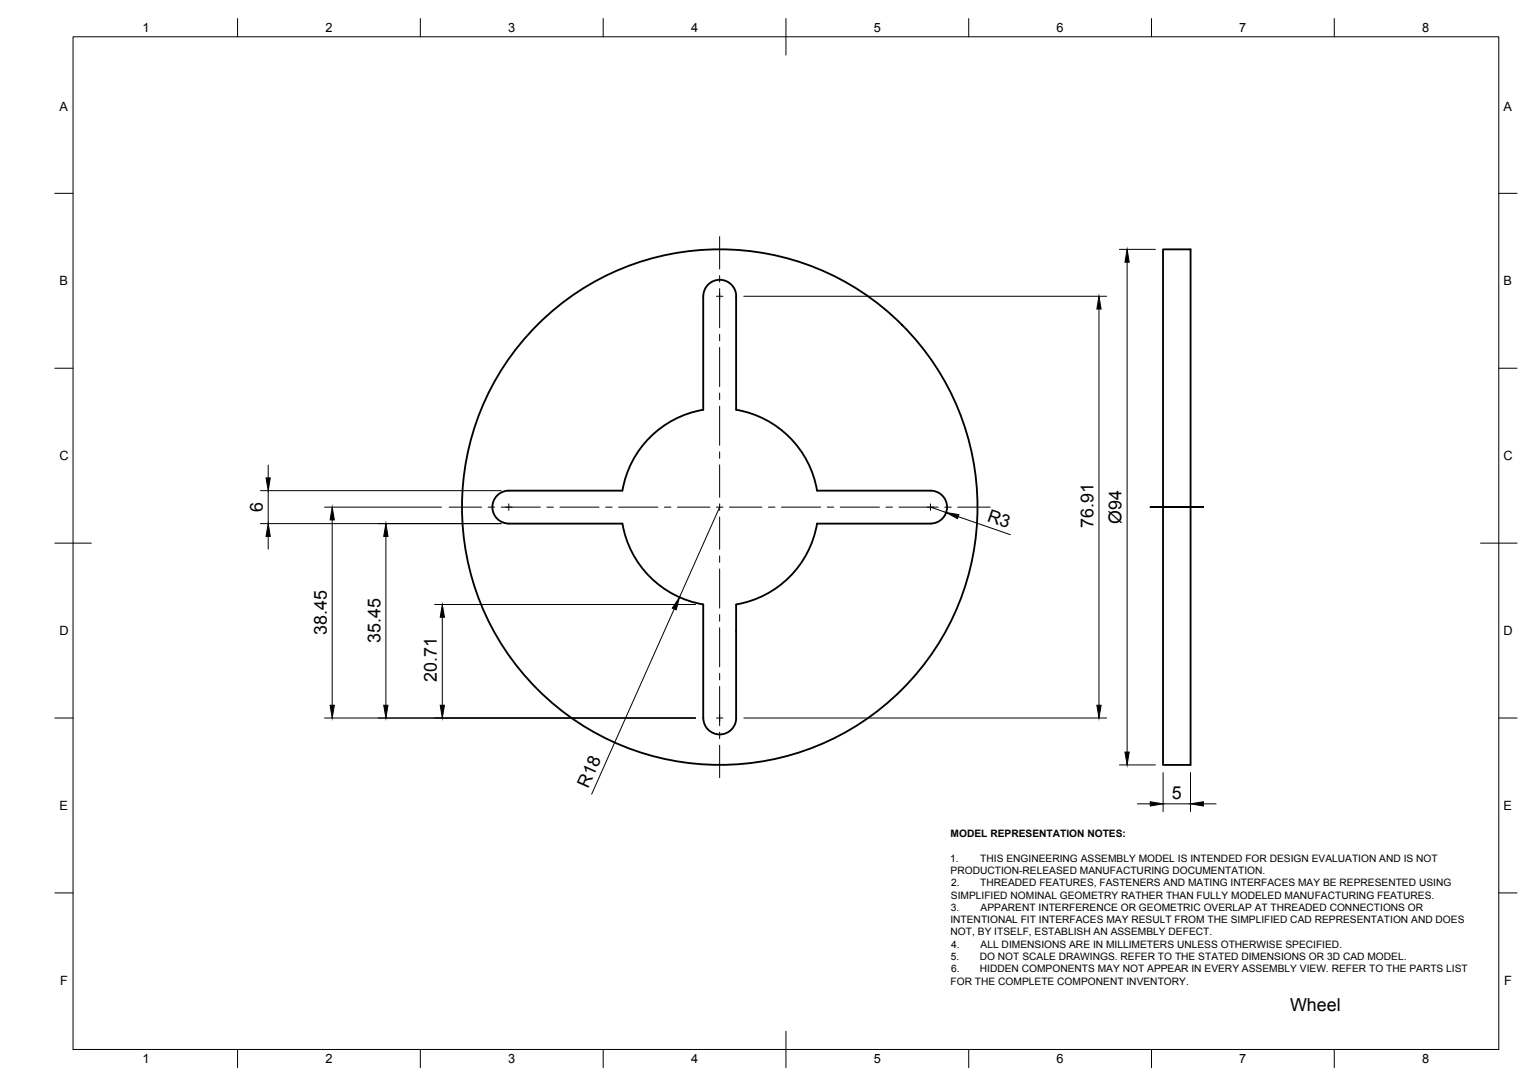
ISO-10303-21;
HEADER;
/* Generated by software containing ST-Developer
 * from STEP Tools, Inc. (www.steptools.com) 
 */

FILE_DESCRIPTION(
/* description */ (''),
/* implementation_level */ '2;1');

FILE_NAME(
/* name */ 'Wheel.step',
/* time_stamp */ '2026-10-04T12:17:52-07:00',
/* author */ (''),
/* organization */ (''),
/* preprocessor_version */ 'ST-DEVELOPER v20.2',
/* originating_system */ 'Autodesk Translation Framework v15.15.0.0',
/* authorisation */ '');

FILE_SCHEMA (('AUTOMOTIVE_DESIGN { 1 0 10303 214 3 1 1 }'));
ENDSEC;

DATA;
#10=MECHANICAL_DESIGN_GEOMETRIC_PRESENTATION_REPRESENTATION('',(#63),#1602);
#47=SHAPE_REPRESENTATION_RELATIONSHIP('SRR','None',#1634,#55);
#55=ADVANCED_BREP_SHAPE_REPRESENTATION('',(#71),#1594);
#63=STYLED_ITEM('',(#1683),#71);
#71=MANIFOLD_SOLID_BREP('Body1',#774);
#79=FACE_BOUND('',#221,.T.);
#80=FACE_BOUND('',#223,.T.);
#93=CIRCLE('',#875,18.);
#94=CIRCLE('',#876,18.);
#95=CIRCLE('',#879,3.);
#96=CIRCLE('',#880,3.);
#97=CIRCLE('',#883,18.);
#98=CIRCLE('',#884,18.);
#99=CIRCLE('',#887,3.);
#100=CIRCLE('',#888,3.);
#101=CIRCLE('',#891,18.);
#102=CIRCLE('',#892,18.);
#103=CIRCLE('',#895,3.);
#104=CIRCLE('',#896,3.);
#105=CIRCLE('',#899,18.);
#106=CIRCLE('',#900,18.);
#107=CIRCLE('',#903,3.);
#108=CIRCLE('',#904,3.);
#109=CIRCLE('',#907,47.);
#110=CIRCLE('',#908,47.);
#133=CYLINDRICAL_SURFACE('',#874,18.);
#134=CYLINDRICAL_SURFACE('',#878,3.);
#135=CYLINDRICAL_SURFACE('',#882,18.);
#136=CYLINDRICAL_SURFACE('',#886,3.);
#137=CYLINDRICAL_SURFACE('',#890,18.);
#138=CYLINDRICAL_SURFACE('',#894,3.);
#139=CYLINDRICAL_SURFACE('',#898,18.);
#140=CYLINDRICAL_SURFACE('',#902,3.);
#141=CYLINDRICAL_SURFACE('',#906,47.);
#155=FACE_OUTER_BOUND('',#202,.T.);
#156=FACE_OUTER_BOUND('',#203,.T.);
#157=FACE_OUTER_BOUND('',#204,.T.);
#158=FACE_OUTER_BOUND('',#205,.T.);
#159=FACE_OUTER_BOUND('',#206,.T.);
#160=FACE_OUTER_BOUND('',#207,.T.);
#161=FACE_OUTER_BOUND('',#208,.T.);
#162=FACE_OUTER_BOUND('',#209,.T.);
#163=FACE_OUTER_BOUND('',#210,.T.);
#164=FACE_OUTER_BOUND('',#211,.T.);
#165=FACE_OUTER_BOUND('',#212,.T.);
#166=FACE_OUTER_BOUND('',#213,.T.);
#167=FACE_OUTER_BOUND('',#214,.T.);
#168=FACE_OUTER_BOUND('',#215,.T.);
#169=FACE_OUTER_BOUND('',#216,.T.);
#170=FACE_OUTER_BOUND('',#217,.T.);
#171=FACE_OUTER_BOUND('',#218,.T.);
#172=FACE_OUTER_BOUND('',#219,.T.);
#173=FACE_OUTER_BOUND('',#220,.T.);
#174=FACE_OUTER_BOUND('',#222,.T.);
#202=EDGE_LOOP('',(#516,#517,#518,#519));
#203=EDGE_LOOP('',(#520,#521,#522,#523));
#204=EDGE_LOOP('',(#524,#525,#526,#527));
#205=EDGE_LOOP('',(#528,#529,#530,#531));
#206=EDGE_LOOP('',(#532,#533,#534,#535));
#207=EDGE_LOOP('',(#536,#537,#538,#539));
#208=EDGE_LOOP('',(#540,#541,#542,#543));
#209=EDGE_LOOP('',(#544,#545,#546,#547));
#210=EDGE_LOOP('',(#548,#549,#550,#551));
#211=EDGE_LOOP('',(#552,#553,#554,#555));
#212=EDGE_LOOP('',(#556,#557,#558,#559));
#213=EDGE_LOOP('',(#560,#561,#562,#563));
#214=EDGE_LOOP('',(#564,#565,#566,#567));
#215=EDGE_LOOP('',(#568,#569,#570,#571));
#216=EDGE_LOOP('',(#572,#573,#574,#575));
#217=EDGE_LOOP('',(#576,#577,#578,#579));
#218=EDGE_LOOP('',(#580,#581,#582,#583));
#219=EDGE_LOOP('',(#584,#585,#586,#587));
#220=EDGE_LOOP('',(#588));
#221=EDGE_LOOP('',(#589,#590,#591,#592,#593,#594,#595,#596,#597,#598,#599,
#600,#601,#602,#603,#604,#605));
#222=EDGE_LOOP('',(#606));
#223=EDGE_LOOP('',(#607,#608,#609,#610,#611,#612,#613,#614,#615,#616,#617,
#618,#619,#620,#621,#622,#623));
#263=LINE('',#1237,#312);
#264=LINE('',#1239,#313);
#265=LINE('',#1241,#314);
#266=LINE('',#1242,#315);
#267=LINE('',#1248,#316);
#268=LINE('',#1251,#317);
#269=LINE('',#1254,#318);
#270=LINE('',#1256,#319);
#271=LINE('',#1257,#320);
#272=LINE('',#1263,#321);
#273=LINE('',#1266,#322);
#274=LINE('',#1268,#323);
#275=LINE('',#1269,#324);
#276=LINE('',#1275,#325);
#277=LINE('',#1278,#326);
#278=LINE('',#1280,#327);
#279=LINE('',#1281,#328);
#280=LINE('',#1287,#329);
#281=LINE('',#1290,#330);
#282=LINE('',#1292,#331);
#283=LINE('',#1293,#332);
#284=LINE('',#1299,#333);
#285=LINE('',#1302,#334);
#286=LINE('',#1304,#335);
#287=LINE('',#1305,#336);
#288=LINE('',#1311,#337);
#289=LINE('',#1314,#338);
#290=LINE('',#1316,#339);
#291=LINE('',#1317,#340);
#292=LINE('',#1323,#341);
#293=LINE('',#1325,#342);
#294=LINE('',#1326,#343);
#295=LINE('',#1332,#344);
#296=LINE('',#1334,#345);
#297=LINE('',#1335,#346);
#298=LINE('',#1340,#347);
#312=VECTOR('',#981,10.);
#313=VECTOR('',#982,10.);
#314=VECTOR('',#983,10.);
#315=VECTOR('',#984,10.);
#316=VECTOR('',#989,10.);
#317=VECTOR('',#992,10.);
#318=VECTOR('',#995,10.);
#319=VECTOR('',#996,10.);
#320=VECTOR('',#997,10.);
#321=VECTOR('',#1004,10.);
#322=VECTOR('',#1007,10.);
#323=VECTOR('',#1008,10.);
#324=VECTOR('',#1009,10.);
#325=VECTOR('',#1016,10.);
#326=VECTOR('',#1019,10.);
#327=VECTOR('',#1020,10.);
#328=VECTOR('',#1021,10.);
#329=VECTOR('',#1028,10.);
#330=VECTOR('',#1031,10.);
#331=VECTOR('',#1032,10.);
#332=VECTOR('',#1033,10.);
#333=VECTOR('',#1040,10.);
#334=VECTOR('',#1043,10.);
#335=VECTOR('',#1044,10.);
#336=VECTOR('',#1045,10.);
#337=VECTOR('',#1052,10.);
#338=VECTOR('',#1055,10.);
#339=VECTOR('',#1056,10.);
#340=VECTOR('',#1057,10.);
#341=VECTOR('',#1066,10.);
#342=VECTOR('',#1067,10.);
#343=VECTOR('',#1068,10.);
#344=VECTOR('',#1075,10.);
#345=VECTOR('',#1078,10.);
#346=VECTOR('',#1079,10.);
#347=VECTOR('',#1084,47.);
#361=VERTEX_POINT('',#1235);
#362=VERTEX_POINT('',#1236);
#363=VERTEX_POINT('',#1238);
#364=VERTEX_POINT('',#1240);
#365=VERTEX_POINT('',#1244);
#366=VERTEX_POINT('',#1245);
#367=VERTEX_POINT('',#1247);
#368=VERTEX_POINT('',#1249);
#369=VERTEX_POINT('',#1253);
#370=VERTEX_POINT('',#1255);
#371=VERTEX_POINT('',#1259);
#372=VERTEX_POINT('',#1261);
#373=VERTEX_POINT('',#1265);
#374=VERTEX_POINT('',#1267);
#375=VERTEX_POINT('',#1271);
#376=VERTEX_POINT('',#1273);
#377=VERTEX_POINT('',#1277);
#378=VERTEX_POINT('',#1279);
#379=VERTEX_POINT('',#1283);
#380=VERTEX_POINT('',#1285);
#381=VERTEX_POINT('',#1289);
#382=VERTEX_POINT('',#1291);
#383=VERTEX_POINT('',#1295);
#384=VERTEX_POINT('',#1297);
#385=VERTEX_POINT('',#1301);
#386=VERTEX_POINT('',#1303);
#387=VERTEX_POINT('',#1307);
#388=VERTEX_POINT('',#1309);
#389=VERTEX_POINT('',#1313);
#390=VERTEX_POINT('',#1315);
#391=VERTEX_POINT('',#1322);
#392=VERTEX_POINT('',#1324);
#393=VERTEX_POINT('',#1328);
#394=VERTEX_POINT('',#1330);
#395=VERTEX_POINT('',#1337);
#396=VERTEX_POINT('',#1339);
#423=EDGE_CURVE('',#361,#362,#263,.T.);
#424=EDGE_CURVE('',#363,#362,#264,.T.);
#425=EDGE_CURVE('',#364,#363,#265,.T.);
#426=EDGE_CURVE('',#361,#364,#266,.T.);
#427=EDGE_CURVE('',#365,#366,#93,.T.);
#428=EDGE_CURVE('',#365,#367,#267,.T.);
#429=EDGE_CURVE('',#368,#367,#94,.T.);
#430=EDGE_CURVE('',#366,#368,#268,.T.);
#431=EDGE_CURVE('',#366,#369,#269,.T.);
#432=EDGE_CURVE('',#370,#368,#270,.T.);
#433=EDGE_CURVE('',#369,#370,#271,.T.);
#434=EDGE_CURVE('',#369,#371,#95,.T.);
#435=EDGE_CURVE('',#372,#370,#96,.T.);
#436=EDGE_CURVE('',#371,#372,#272,.T.);
#437=EDGE_CURVE('',#371,#373,#273,.T.);
#438=EDGE_CURVE('',#374,#372,#274,.T.);
#439=EDGE_CURVE('',#374,#373,#275,.T.);
#440=EDGE_CURVE('',#373,#375,#97,.T.);
#441=EDGE_CURVE('',#374,#376,#98,.T.);
#442=EDGE_CURVE('',#375,#376,#276,.T.);
#443=EDGE_CURVE('',#375,#377,#277,.T.);
#444=EDGE_CURVE('',#378,#376,#278,.T.);
#445=EDGE_CURVE('',#377,#378,#279,.T.);
#446=EDGE_CURVE('',#377,#379,#99,.T.);
#447=EDGE_CURVE('',#380,#378,#100,.T.);
#448=EDGE_CURVE('',#379,#380,#280,.T.);
#449=EDGE_CURVE('',#379,#381,#281,.T.);
#450=EDGE_CURVE('',#382,#380,#282,.T.);
#451=EDGE_CURVE('',#381,#382,#283,.T.);
#452=EDGE_CURVE('',#381,#383,#101,.T.);
#453=EDGE_CURVE('',#384,#382,#102,.T.);
#454=EDGE_CURVE('',#383,#384,#284,.T.);
#455=EDGE_CURVE('',#383,#385,#285,.T.);
#456=EDGE_CURVE('',#386,#384,#286,.T.);
#457=EDGE_CURVE('',#385,#386,#287,.T.);
#458=EDGE_CURVE('',#385,#387,#103,.T.);
#459=EDGE_CURVE('',#388,#386,#104,.T.);
#460=EDGE_CURVE('',#387,#388,#288,.T.);
#461=EDGE_CURVE('',#387,#389,#289,.T.);
#462=EDGE_CURVE('',#390,#388,#290,.T.);
#463=EDGE_CURVE('',#389,#390,#291,.T.);
#464=EDGE_CURVE('',#389,#362,#105,.T.);
#465=EDGE_CURVE('',#363,#390,#106,.T.);
#466=EDGE_CURVE('',#361,#391,#292,.T.);
#467=EDGE_CURVE('',#392,#364,#293,.T.);
#468=EDGE_CURVE('',#391,#392,#294,.T.);
#469=EDGE_CURVE('',#391,#393,#107,.T.);
#470=EDGE_CURVE('',#394,#392,#108,.T.);
#471=EDGE_CURVE('',#393,#394,#295,.T.);
#472=EDGE_CURVE('',#393,#365,#296,.T.);
#473=EDGE_CURVE('',#367,#394,#297,.T.);
#474=EDGE_CURVE('',#395,#395,#109,.T.);
#475=EDGE_CURVE('',#395,#396,#298,.T.);
#476=EDGE_CURVE('',#396,#396,#110,.T.);
#516=ORIENTED_EDGE('',*,*,#423,.T.);
#517=ORIENTED_EDGE('',*,*,#424,.F.);
#518=ORIENTED_EDGE('',*,*,#425,.F.);
#519=ORIENTED_EDGE('',*,*,#426,.F.);
#520=ORIENTED_EDGE('',*,*,#427,.F.);
#521=ORIENTED_EDGE('',*,*,#428,.T.);
#522=ORIENTED_EDGE('',*,*,#429,.F.);
#523=ORIENTED_EDGE('',*,*,#430,.F.);
#524=ORIENTED_EDGE('',*,*,#431,.F.);
#525=ORIENTED_EDGE('',*,*,#430,.T.);
#526=ORIENTED_EDGE('',*,*,#432,.F.);
#527=ORIENTED_EDGE('',*,*,#433,.F.);
#528=ORIENTED_EDGE('',*,*,#434,.F.);
#529=ORIENTED_EDGE('',*,*,#433,.T.);
#530=ORIENTED_EDGE('',*,*,#435,.F.);
#531=ORIENTED_EDGE('',*,*,#436,.F.);
#532=ORIENTED_EDGE('',*,*,#437,.F.);
#533=ORIENTED_EDGE('',*,*,#436,.T.);
#534=ORIENTED_EDGE('',*,*,#438,.F.);
#535=ORIENTED_EDGE('',*,*,#439,.T.);
#536=ORIENTED_EDGE('',*,*,#440,.F.);
#537=ORIENTED_EDGE('',*,*,#439,.F.);
#538=ORIENTED_EDGE('',*,*,#441,.T.);
#539=ORIENTED_EDGE('',*,*,#442,.F.);
#540=ORIENTED_EDGE('',*,*,#443,.F.);
#541=ORIENTED_EDGE('',*,*,#442,.T.);
#542=ORIENTED_EDGE('',*,*,#444,.F.);
#543=ORIENTED_EDGE('',*,*,#445,.F.);
#544=ORIENTED_EDGE('',*,*,#446,.F.);
#545=ORIENTED_EDGE('',*,*,#445,.T.);
#546=ORIENTED_EDGE('',*,*,#447,.F.);
#547=ORIENTED_EDGE('',*,*,#448,.F.);
#548=ORIENTED_EDGE('',*,*,#449,.F.);
#549=ORIENTED_EDGE('',*,*,#448,.T.);
#550=ORIENTED_EDGE('',*,*,#450,.F.);
#551=ORIENTED_EDGE('',*,*,#451,.F.);
#552=ORIENTED_EDGE('',*,*,#452,.F.);
#553=ORIENTED_EDGE('',*,*,#451,.T.);
#554=ORIENTED_EDGE('',*,*,#453,.F.);
#555=ORIENTED_EDGE('',*,*,#454,.F.);
#556=ORIENTED_EDGE('',*,*,#455,.F.);
#557=ORIENTED_EDGE('',*,*,#454,.T.);
#558=ORIENTED_EDGE('',*,*,#456,.F.);
#559=ORIENTED_EDGE('',*,*,#457,.F.);
#560=ORIENTED_EDGE('',*,*,#458,.F.);
#561=ORIENTED_EDGE('',*,*,#457,.T.);
#562=ORIENTED_EDGE('',*,*,#459,.F.);
#563=ORIENTED_EDGE('',*,*,#460,.F.);
#564=ORIENTED_EDGE('',*,*,#461,.F.);
#565=ORIENTED_EDGE('',*,*,#460,.T.);
#566=ORIENTED_EDGE('',*,*,#462,.F.);
#567=ORIENTED_EDGE('',*,*,#463,.F.);
#568=ORIENTED_EDGE('',*,*,#464,.F.);
#569=ORIENTED_EDGE('',*,*,#463,.T.);
#570=ORIENTED_EDGE('',*,*,#465,.F.);
#571=ORIENTED_EDGE('',*,*,#424,.T.);
#572=ORIENTED_EDGE('',*,*,#466,.F.);
#573=ORIENTED_EDGE('',*,*,#426,.T.);
#574=ORIENTED_EDGE('',*,*,#467,.F.);
#575=ORIENTED_EDGE('',*,*,#468,.F.);
#576=ORIENTED_EDGE('',*,*,#469,.F.);
#577=ORIENTED_EDGE('',*,*,#468,.T.);
#578=ORIENTED_EDGE('',*,*,#470,.F.);
#579=ORIENTED_EDGE('',*,*,#471,.F.);
#580=ORIENTED_EDGE('',*,*,#472,.F.);
#581=ORIENTED_EDGE('',*,*,#471,.T.);
#582=ORIENTED_EDGE('',*,*,#473,.F.);
#583=ORIENTED_EDGE('',*,*,#428,.F.);
#584=ORIENTED_EDGE('',*,*,#474,.F.);
#585=ORIENTED_EDGE('',*,*,#475,.T.);
#586=ORIENTED_EDGE('',*,*,#476,.F.);
#587=ORIENTED_EDGE('',*,*,#475,.F.);
#588=ORIENTED_EDGE('',*,*,#476,.T.);
#589=ORIENTED_EDGE('',*,*,#472,.T.);
#590=ORIENTED_EDGE('',*,*,#427,.T.);
#591=ORIENTED_EDGE('',*,*,#431,.T.);
#592=ORIENTED_EDGE('',*,*,#434,.T.);
#593=ORIENTED_EDGE('',*,*,#437,.T.);
#594=ORIENTED_EDGE('',*,*,#440,.T.);
#595=ORIENTED_EDGE('',*,*,#443,.T.);
#596=ORIENTED_EDGE('',*,*,#446,.T.);
#597=ORIENTED_EDGE('',*,*,#449,.T.);
#598=ORIENTED_EDGE('',*,*,#452,.T.);
#599=ORIENTED_EDGE('',*,*,#455,.T.);
#600=ORIENTED_EDGE('',*,*,#458,.T.);
#601=ORIENTED_EDGE('',*,*,#461,.T.);
#602=ORIENTED_EDGE('',*,*,#464,.T.);
#603=ORIENTED_EDGE('',*,*,#423,.F.);
#604=ORIENTED_EDGE('',*,*,#466,.T.);
#605=ORIENTED_EDGE('',*,*,#469,.T.);
#606=ORIENTED_EDGE('',*,*,#474,.T.);
#607=ORIENTED_EDGE('',*,*,#473,.T.);
#608=ORIENTED_EDGE('',*,*,#470,.T.);
#609=ORIENTED_EDGE('',*,*,#467,.T.);
#610=ORIENTED_EDGE('',*,*,#425,.T.);
#611=ORIENTED_EDGE('',*,*,#465,.T.);
#612=ORIENTED_EDGE('',*,*,#462,.T.);
#613=ORIENTED_EDGE('',*,*,#459,.T.);
#614=ORIENTED_EDGE('',*,*,#456,.T.);
#615=ORIENTED_EDGE('',*,*,#453,.T.);
#616=ORIENTED_EDGE('',*,*,#450,.T.);
#617=ORIENTED_EDGE('',*,*,#447,.T.);
#618=ORIENTED_EDGE('',*,*,#444,.T.);
#619=ORIENTED_EDGE('',*,*,#441,.F.);
#620=ORIENTED_EDGE('',*,*,#438,.T.);
#621=ORIENTED_EDGE('',*,*,#435,.T.);
#622=ORIENTED_EDGE('',*,*,#432,.T.);
#623=ORIENTED_EDGE('',*,*,#429,.T.);
#702=PLANE('',#873);
#703=PLANE('',#877);
#704=PLANE('',#881);
#705=PLANE('',#885);
#706=PLANE('',#889);
#707=PLANE('',#893);
#708=PLANE('',#897);
#709=PLANE('',#901);
#710=PLANE('',#905);
#711=PLANE('',#909);
#712=PLANE('',#910);
#727=ADVANCED_FACE('',(#155),#702,.T.);
#728=ADVANCED_FACE('',(#156),#133,.F.);
#729=ADVANCED_FACE('',(#157),#703,.T.);
#730=ADVANCED_FACE('',(#158),#134,.F.);
#731=ADVANCED_FACE('',(#159),#704,.T.);
#732=ADVANCED_FACE('',(#160),#135,.F.);
#733=ADVANCED_FACE('',(#161),#705,.T.);
#734=ADVANCED_FACE('',(#162),#136,.F.);
#735=ADVANCED_FACE('',(#163),#706,.T.);
#736=ADVANCED_FACE('',(#164),#137,.F.);
#737=ADVANCED_FACE('',(#165),#707,.T.);
#738=ADVANCED_FACE('',(#166),#138,.F.);
#739=ADVANCED_FACE('',(#167),#708,.T.);
#740=ADVANCED_FACE('',(#168),#139,.F.);
#741=ADVANCED_FACE('',(#169),#709,.T.);
#742=ADVANCED_FACE('',(#170),#140,.F.);
#743=ADVANCED_FACE('',(#171),#710,.T.);
#744=ADVANCED_FACE('',(#172),#141,.T.);
#745=ADVANCED_FACE('',(#173,#79),#711,.T.);
#746=ADVANCED_FACE('',(#174,#80),#712,.F.);
#774=CLOSED_SHELL('',(#727,#728,#729,#730,#731,#732,#733,#734,#735,#736,
#737,#738,#739,#740,#741,#742,#743,#744,#745,#746));
#872=AXIS2_PLACEMENT_3D('',#1233,#977,#978);
#873=AXIS2_PLACEMENT_3D('',#1234,#979,#980);
#874=AXIS2_PLACEMENT_3D('',#1243,#985,#986);
#875=AXIS2_PLACEMENT_3D('',#1246,#987,#988);
#876=AXIS2_PLACEMENT_3D('',#1250,#990,#991);
#877=AXIS2_PLACEMENT_3D('',#1252,#993,#994);
#878=AXIS2_PLACEMENT_3D('',#1258,#998,#999);
#879=AXIS2_PLACEMENT_3D('',#1260,#1000,#1001);
#880=AXIS2_PLACEMENT_3D('',#1262,#1002,#1003);
#881=AXIS2_PLACEMENT_3D('',#1264,#1005,#1006);
#882=AXIS2_PLACEMENT_3D('',#1270,#1010,#1011);
#883=AXIS2_PLACEMENT_3D('',#1272,#1012,#1013);
#884=AXIS2_PLACEMENT_3D('',#1274,#1014,#1015);
#885=AXIS2_PLACEMENT_3D('',#1276,#1017,#1018);
#886=AXIS2_PLACEMENT_3D('',#1282,#1022,#1023);
#887=AXIS2_PLACEMENT_3D('',#1284,#1024,#1025);
#888=AXIS2_PLACEMENT_3D('',#1286,#1026,#1027);
#889=AXIS2_PLACEMENT_3D('',#1288,#1029,#1030);
#890=AXIS2_PLACEMENT_3D('',#1294,#1034,#1035);
#891=AXIS2_PLACEMENT_3D('',#1296,#1036,#1037);
#892=AXIS2_PLACEMENT_3D('',#1298,#1038,#1039);
#893=AXIS2_PLACEMENT_3D('',#1300,#1041,#1042);
#894=AXIS2_PLACEMENT_3D('',#1306,#1046,#1047);
#895=AXIS2_PLACEMENT_3D('',#1308,#1048,#1049);
#896=AXIS2_PLACEMENT_3D('',#1310,#1050,#1051);
#897=AXIS2_PLACEMENT_3D('',#1312,#1053,#1054);
#898=AXIS2_PLACEMENT_3D('',#1318,#1058,#1059);
#899=AXIS2_PLACEMENT_3D('',#1319,#1060,#1061);
#900=AXIS2_PLACEMENT_3D('',#1320,#1062,#1063);
#901=AXIS2_PLACEMENT_3D('',#1321,#1064,#1065);
#902=AXIS2_PLACEMENT_3D('',#1327,#1069,#1070);
#903=AXIS2_PLACEMENT_3D('',#1329,#1071,#1072);
#904=AXIS2_PLACEMENT_3D('',#1331,#1073,#1074);
#905=AXIS2_PLACEMENT_3D('',#1333,#1076,#1077);
#906=AXIS2_PLACEMENT_3D('',#1336,#1080,#1081);
#907=AXIS2_PLACEMENT_3D('',#1338,#1082,#1083);
#908=AXIS2_PLACEMENT_3D('',#1341,#1085,#1086);
#909=AXIS2_PLACEMENT_3D('',#1342,#1087,#1088);
#910=AXIS2_PLACEMENT_3D('',#1343,#1089,#1090);
#977=DIRECTION('axis',(0.,0.,1.));
#978=DIRECTION('refdir',(1.,0.,0.));
#979=DIRECTION('center_axis',(0.707106813733351,0.,0.707106748639742));
#980=DIRECTION('ref_axis',(0.707106748639742,0.,-0.707106813733351));
#981=DIRECTION('',(-0.707106748639742,0.,0.707106813733351));
#982=DIRECTION('',(0.,1.,0.));
#983=DIRECTION('',(-0.707106748639742,0.,0.707106813733351));
#984=DIRECTION('',(0.,-1.,0.));
#985=DIRECTION('center_axis',(0.,-1.,0.));
#986=DIRECTION('ref_axis',(1.,0.,0.));
#987=DIRECTION('center_axis',(0.,-1.,0.));
#988=DIRECTION('ref_axis',(1.,0.,0.));
#989=DIRECTION('',(0.,-1.,0.));
#990=DIRECTION('center_axis',(0.,1.,0.));
#991=DIRECTION('ref_axis',(1.,0.,0.));
#992=DIRECTION('',(0.,-1.,0.));
#993=DIRECTION('center_axis',(-0.707106781186548,0.,0.707106781186547));
#994=DIRECTION('ref_axis',(-0.707106781186547,0.,-0.707106781186548));
#995=DIRECTION('',(0.707106781186547,0.,0.707106781186548));
#996=DIRECTION('',(-0.707106781186547,0.,-0.707106781186548));
#997=DIRECTION('',(0.,-1.,0.));
#998=DIRECTION('center_axis',(0.,-1.,0.));
#999=DIRECTION('ref_axis',(-0.707106781186549,0.,0.707106781186546));
#1000=DIRECTION('center_axis',(0.,-1.,0.));
#1001=DIRECTION('ref_axis',(-0.707106781186549,0.,0.707106781186546));
#1002=DIRECTION('center_axis',(0.,1.,0.));
#1003=DIRECTION('ref_axis',(-0.707106781186549,0.,0.707106781186546));
#1004=DIRECTION('',(0.,-1.,0.));
#1005=DIRECTION('center_axis',(0.707106781186548,0.,-0.707106781186548));
#1006=DIRECTION('ref_axis',(0.707106781186548,0.,0.707106781186548));
#1007=DIRECTION('',(-0.707106781186547,0.,-0.707106781186547));
#1008=DIRECTION('',(0.707106781186547,0.,0.707106781186547));
#1009=DIRECTION('',(0.,1.,0.));
#1010=DIRECTION('center_axis',(0.,-1.,0.));
#1011=DIRECTION('ref_axis',(1.,0.,0.));
#1012=DIRECTION('center_axis',(0.,-1.,0.));
#1013=DIRECTION('ref_axis',(1.,0.,0.));
#1014=DIRECTION('center_axis',(0.,-1.,0.));
#1015=DIRECTION('ref_axis',(0.579365558580642,0.,0.815067818976151));
#1016=DIRECTION('',(0.,-1.,0.));
#1017=DIRECTION('center_axis',(-0.707106781186548,0.,-0.707106781186547));
#1018=DIRECTION('ref_axis',(0.707106781186547,0.,-0.707106781186548));
#1019=DIRECTION('',(-0.707106781186547,0.,0.707106781186548));
#1020=DIRECTION('',(0.707106781186547,0.,-0.707106781186548));
#1021=DIRECTION('',(0.,-1.,0.));
#1022=DIRECTION('center_axis',(0.,-1.,0.));
#1023=DIRECTION('ref_axis',(-0.707106781186547,0.,-0.707106781186548));
#1024=DIRECTION('center_axis',(0.,-1.,0.));
#1025=DIRECTION('ref_axis',(-0.707106781186547,0.,-0.707106781186548));
#1026=DIRECTION('center_axis',(0.,1.,0.));
#1027=DIRECTION('ref_axis',(-0.707106781186547,0.,-0.707106781186548));
#1028=DIRECTION('',(0.,-1.,0.));
#1029=DIRECTION('center_axis',(0.707106781186548,0.,0.707106781186547));
#1030=DIRECTION('ref_axis',(-0.707106781186547,0.,0.707106781186548));
#1031=DIRECTION('',(0.707106781186547,0.,-0.707106781186548));
#1032=DIRECTION('',(-0.707106781186547,0.,0.707106781186548));
#1033=DIRECTION('',(0.,-1.,0.));
#1034=DIRECTION('center_axis',(0.,-1.,0.));
#1035=DIRECTION('ref_axis',(-1.,0.,1.22464679914735E-16));
#1036=DIRECTION('center_axis',(0.,-1.,0.));
#1037=DIRECTION('ref_axis',(1.,0.,0.));
#1038=DIRECTION('center_axis',(0.,1.,0.));
#1039=DIRECTION('ref_axis',(1.,0.,0.));
#1040=DIRECTION('',(0.,-1.,0.));
#1041=DIRECTION('center_axis',(0.707106781186547,0.,-0.707106781186548));
#1042=DIRECTION('ref_axis',(0.707106781186548,0.,0.707106781186547));
#1043=DIRECTION('',(-0.707106781186548,0.,-0.707106781186547));
#1044=DIRECTION('',(0.707106781186548,0.,0.707106781186547));
#1045=DIRECTION('',(0.,-1.,0.));
#1046=DIRECTION('center_axis',(0.,-1.,0.));
#1047=DIRECTION('ref_axis',(-0.707106786454903,0.,-0.707106775918192));
#1048=DIRECTION('center_axis',(0.,-1.,0.));
#1049=DIRECTION('ref_axis',(0.707106781186548,0.,-0.707106781186547));
#1050=DIRECTION('center_axis',(0.,1.,0.));
#1051=DIRECTION('ref_axis',(0.707106781186548,0.,-0.707106781186547));
#1052=DIRECTION('',(0.,-1.,0.));
#1053=DIRECTION('center_axis',(-0.707106781186547,0.,0.707106781186548));
#1054=DIRECTION('ref_axis',(-0.707106781186548,0.,-0.707106781186547));
#1055=DIRECTION('',(0.707106781186548,0.,0.707106781186547));
#1056=DIRECTION('',(-0.707106781186548,0.,-0.707106781186547));
#1057=DIRECTION('',(0.,-1.,0.));
#1058=DIRECTION('center_axis',(0.,-1.,0.));
#1059=DIRECTION('ref_axis',(1.,0.,0.));
#1060=DIRECTION('center_axis',(0.,-1.,0.));
#1061=DIRECTION('ref_axis',(1.,0.,0.));
#1062=DIRECTION('center_axis',(0.,1.,0.));
#1063=DIRECTION('ref_axis',(1.,0.,0.));
#1064=DIRECTION('center_axis',(0.707106781186548,0.,0.707106781186547));
#1065=DIRECTION('ref_axis',(-0.707106781186547,0.,0.707106781186548));
#1066=DIRECTION('',(0.707106781186547,0.,-0.707106781186548));
#1067=DIRECTION('',(-0.707106781186547,0.,0.707106781186548));
#1068=DIRECTION('',(0.,-1.,0.));
#1069=DIRECTION('center_axis',(0.,-1.,0.));
#1070=DIRECTION('ref_axis',(0.707106775918192,0.,-0.707106786454903));
#1071=DIRECTION('center_axis',(0.,-1.,0.));
#1072=DIRECTION('ref_axis',(0.707106781186547,0.,0.707106781186548));
#1073=DIRECTION('center_axis',(0.,1.,0.));
#1074=DIRECTION('ref_axis',(0.707106781186547,0.,0.707106781186548));
#1075=DIRECTION('',(0.,-1.,0.));
#1076=DIRECTION('center_axis',(-0.707106781186548,0.,-0.707106781186547));
#1077=DIRECTION('ref_axis',(0.707106781186547,0.,-0.707106781186548));
#1078=DIRECTION('',(-0.707106781186547,0.,0.707106781186548));
#1079=DIRECTION('',(0.707106781186547,0.,-0.707106781186548));
#1080=DIRECTION('center_axis',(0.,-1.,0.));
#1081=DIRECTION('ref_axis',(1.,0.,0.));
#1082=DIRECTION('center_axis',(0.,-1.,0.));
#1083=DIRECTION('ref_axis',(1.,0.,0.));
#1084=DIRECTION('',(0.,1.,0.));
#1085=DIRECTION('center_axis',(0.,1.,0.));
#1086=DIRECTION('ref_axis',(1.,0.,0.));
#1087=DIRECTION('center_axis',(0.,1.,0.));
#1088=DIRECTION('ref_axis',(1.,0.,0.));
#1089=DIRECTION('center_axis',(0.,1.,0.));
#1090=DIRECTION('ref_axis',(1.,0.,0.));
#1233=CARTESIAN_POINT('',(0.,0.,0.));
#1234=CARTESIAN_POINT('Origin',(10.4285802387844,-8.,35.3287793894565));
#1235=CARTESIAN_POINT('',(13.854312705131,-3.,31.9030466077497));
#1236=CARTESIAN_POINT('',(10.4285802387843,-3.,35.3287793894565));
#1237=CARTESIAN_POINT('',(7.10531883627285,-3.,38.6520410978951));
#1238=CARTESIAN_POINT('',(10.4285802387843,-8.,35.3287793894565));
#1239=CARTESIAN_POINT('',(10.4285802387843,-8.,35.3287793894565));
#1240=CARTESIAN_POINT('',(13.854312705131,-8.,31.9030466077497));
#1241=CARTESIAN_POINT('',(13.854312705131,-8.,31.9030466077497));
#1242=CARTESIAN_POINT('',(13.854312705131,-3.,31.9030466077497));
#1243=CARTESIAN_POINT('Origin',(0.,-3.,50.));
#1244=CARTESIAN_POINT('',(14.6712207415708,-3.,39.5714199455485));
#1245=CARTESIAN_POINT('',(14.6712207415708,-3.,60.4285800544515));
#1246=CARTESIAN_POINT('Origin',(0.,-3.,50.));
#1247=CARTESIAN_POINT('',(14.6712207415708,-8.,39.5714199455485));
#1248=CARTESIAN_POINT('',(14.6712207415708,-3.,39.5714199455485));
#1249=CARTESIAN_POINT('',(14.6712207415708,-8.,60.4285800544515));
#1250=CARTESIAN_POINT('Origin',(0.,-8.,50.));
#1251=CARTESIAN_POINT('',(14.6712207415708,-3.,60.4285800544515));
#1252=CARTESIAN_POINT('Origin',(29.3122930478506,-3.,75.0696523607313));
#1253=CARTESIAN_POINT('',(29.3122930478506,-3.,75.0696523607313));
#1254=CARTESIAN_POINT('',(29.3122930478506,-3.,75.0696523607313));
#1255=CARTESIAN_POINT('',(29.3122930478506,-8.,75.0696523607313));
#1256=CARTESIAN_POINT('',(29.3122930478506,-8.,75.0696523607313));
#1257=CARTESIAN_POINT('',(29.3122930478506,-3.,75.0696523607313));
#1258=CARTESIAN_POINT('Origin',(27.190972704291,-3.,77.190972704291));
#1259=CARTESIAN_POINT('',(25.0696523607313,-3.,79.3122930478506));
#1260=CARTESIAN_POINT('Origin',(27.190972704291,-3.,77.190972704291));
#1261=CARTESIAN_POINT('',(25.0696523607313,-8.,79.3122930478506));
#1262=CARTESIAN_POINT('Origin',(27.190972704291,-8.,77.190972704291));
#1263=CARTESIAN_POINT('',(25.0696523607313,-3.,79.3122930478506));
#1264=CARTESIAN_POINT('Origin',(13.854312705131,-3.,68.0969533922503));
#1265=CARTESIAN_POINT('',(10.4285800544516,-3.,64.6712207415707));
#1266=CARTESIAN_POINT('',(6.12338976254612,-3.,60.3660304496654));
#1267=CARTESIAN_POINT('',(10.4285800544516,-8.,64.6712207415707));
#1268=CARTESIAN_POINT('',(6.12338976254612,-8.,60.3660304496654));
#1269=CARTESIAN_POINT('',(10.4285800544516,-8.,64.6712207415707));
#1270=CARTESIAN_POINT('Origin',(0.,-3.,50.));
#1271=CARTESIAN_POINT('',(-10.4285800544515,-3.,64.6712207415708));
#1272=CARTESIAN_POINT('Origin',(0.,-3.,50.));
#1273=CARTESIAN_POINT('',(-10.4285800544515,-8.,64.6712207415708));
#1274=CARTESIAN_POINT('Origin',(0.,-8.,50.));
#1275=CARTESIAN_POINT('',(-10.4285800544515,-3.,64.6712207415708));
#1276=CARTESIAN_POINT('Origin',(-25.0696523607313,-3.,79.3122930478506));
#1277=CARTESIAN_POINT('',(-25.0696523923415,-3.,79.3122930794607));
#1278=CARTESIAN_POINT('',(-25.0696523607313,-3.,79.3122930478506));
#1279=CARTESIAN_POINT('',(-25.0696523923415,-8.,79.3122930794608));
#1280=CARTESIAN_POINT('',(-25.0696523607313,-8.,79.3122930478506));
#1281=CARTESIAN_POINT('',(-25.0696523923415,-3.,79.3122930794607));
#1282=CARTESIAN_POINT('Origin',(-27.190972704291,-3.,77.190972704291));
#1283=CARTESIAN_POINT('',(-29.3122930478506,-3.,75.0696523607313));
#1284=CARTESIAN_POINT('Origin',(-27.190972704291,-3.,77.190972704291));
#1285=CARTESIAN_POINT('',(-29.3122930478506,-8.,75.0696523607313));
#1286=CARTESIAN_POINT('Origin',(-27.190972704291,-8.,77.190972704291));
#1287=CARTESIAN_POINT('',(-29.3122930478506,-3.,75.0696523607313));
#1288=CARTESIAN_POINT('Origin',(-14.6712207415708,-3.,60.4285800544515));
#1289=CARTESIAN_POINT('',(-14.6712207415708,-3.,60.4285800544515));
#1290=CARTESIAN_POINT('',(-10.3660304496654,-3.,56.1233897625461));
#1291=CARTESIAN_POINT('',(-14.6712207415708,-8.,60.4285800544515));
#1292=CARTESIAN_POINT('',(-10.3660304496654,-8.,56.1233897625461));
#1293=CARTESIAN_POINT('',(-14.6712207415708,-3.,60.4285800544515));
#1294=CARTESIAN_POINT('Origin',(0.,-3.,50.));
#1295=CARTESIAN_POINT('',(-14.6712207415708,-3.,39.5714199455485));
#1296=CARTESIAN_POINT('Origin',(0.,-3.,50.));
#1297=CARTESIAN_POINT('',(-14.6712207415708,-8.,39.5714199455485));
#1298=CARTESIAN_POINT('Origin',(0.,-8.,50.));
#1299=CARTESIAN_POINT('',(-14.6712207415708,-3.,39.5714199455485));
#1300=CARTESIAN_POINT('Origin',(-29.3122930162405,-3.,24.9303476708788));
#1301=CARTESIAN_POINT('',(-29.3122930162405,-3.,24.9303476708788));
#1302=CARTESIAN_POINT('',(-29.3122930478506,-3.,24.9303476392687));
#1303=CARTESIAN_POINT('',(-29.3122930162405,-8.,24.9303476708788));
#1304=CARTESIAN_POINT('',(-29.3122930478506,-8.,24.9303476392687));
#1305=CARTESIAN_POINT('',(-29.3122930162405,-3.,24.9303476708788));
#1306=CARTESIAN_POINT('Origin',(-27.190972704291,-3.,22.809027295709));
#1307=CARTESIAN_POINT('',(-25.0696523607313,-3.,20.6877069521494));
#1308=CARTESIAN_POINT('Origin',(-27.190972704291,-3.,22.809027295709));
#1309=CARTESIAN_POINT('',(-25.0696523607313,-8.,20.6877069521494));
#1310=CARTESIAN_POINT('Origin',(-27.190972704291,-8.,22.809027295709));
#1311=CARTESIAN_POINT('',(-25.0696523607313,-3.,20.6877069521494));
#1312=CARTESIAN_POINT('Origin',(-10.4285800544515,-3.,35.3287792584292));
#1313=CARTESIAN_POINT('',(-10.4285800544515,-3.,35.3287792584292));
#1314=CARTESIAN_POINT('',(-6.12338976254612,-3.,39.6339695503346));
#1315=CARTESIAN_POINT('',(-10.4285800544515,-8.,35.3287792584292));
#1316=CARTESIAN_POINT('',(-6.12338976254612,-8.,39.6339695503346));
#1317=CARTESIAN_POINT('',(-10.4285800544515,-3.,35.3287792584292));
#1318=CARTESIAN_POINT('Origin',(0.,-3.,50.));
#1319=CARTESIAN_POINT('Origin',(0.,-3.,50.));
#1320=CARTESIAN_POINT('Origin',(0.,-8.,50.));
#1321=CARTESIAN_POINT('Origin',(25.0696523291212,-3.,20.6877069837595));
#1322=CARTESIAN_POINT('',(25.0696523291212,-3.,20.6877069837595));
#1323=CARTESIAN_POINT('',(25.0696523607313,-3.,20.6877069521494));
#1324=CARTESIAN_POINT('',(25.0696523291212,-8.,20.6877069837595));
#1325=CARTESIAN_POINT('',(25.0696523607313,-8.,20.6877069521494));
#1326=CARTESIAN_POINT('',(25.0696523291212,-3.,20.6877069837595));
#1327=CARTESIAN_POINT('Origin',(27.190972704291,-3.,22.809027295709));
#1328=CARTESIAN_POINT('',(29.3122930478506,-3.,24.9303476392687));
#1329=CARTESIAN_POINT('Origin',(27.190972704291,-3.,22.809027295709));
#1330=CARTESIAN_POINT('',(29.3122930478506,-8.,24.9303476392687));
#1331=CARTESIAN_POINT('Origin',(27.190972704291,-8.,22.809027295709));
#1332=CARTESIAN_POINT('',(29.3122930478506,-3.,24.9303476392687));
#1333=CARTESIAN_POINT('Origin',(14.6712207415708,-3.,39.5714199455485));
#1334=CARTESIAN_POINT('',(10.3660304496654,-3.,43.8766102374539));
#1335=CARTESIAN_POINT('',(10.3660304496654,-8.,43.8766102374539));
#1336=CARTESIAN_POINT('Origin',(0.,-3.,50.));
#1337=CARTESIAN_POINT('',(-47.,-8.,50.));
#1338=CARTESIAN_POINT('Origin',(0.,-8.,50.));
#1339=CARTESIAN_POINT('',(-47.,-3.,50.));
#1340=CARTESIAN_POINT('',(-47.,-3.,50.));
#1341=CARTESIAN_POINT('Origin',(0.,-3.,50.));
#1342=CARTESIAN_POINT('Origin',(0.,-3.,50.));
#1343=CARTESIAN_POINT('Origin',(0.,-8.,50.));
#1584=UNCERTAINTY_MEASURE_WITH_UNIT(LENGTH_MEASURE(0.01),#1603,
'DISTANCE_ACCURACY_VALUE',
'Maximum model space distance between geometric entities at asserted c
onnectivities');
#1592=UNCERTAINTY_MEASURE_WITH_UNIT(LENGTH_MEASURE(0.01),#1603,
'DISTANCE_ACCURACY_VALUE',
'Maximum model space distance between geometric entities at asserted c
onnectivities');
#1594=(
GEOMETRIC_REPRESENTATION_CONTEXT(3)
GLOBAL_UNCERTAINTY_ASSIGNED_CONTEXT((#1584))
GLOBAL_UNIT_ASSIGNED_CONTEXT((#1603,#1605,#1606))
REPRESENTATION_CONTEXT('','3D')
);
#1602=(
GEOMETRIC_REPRESENTATION_CONTEXT(3)
GLOBAL_UNCERTAINTY_ASSIGNED_CONTEXT((#1592))
GLOBAL_UNIT_ASSIGNED_CONTEXT((#1603,#1605,#1606))
REPRESENTATION_CONTEXT('','3D')
);
#1603=(
LENGTH_UNIT()
NAMED_UNIT(*)
SI_UNIT(.MILLI.,.METRE.)
);
#1605=(
NAMED_UNIT(*)
PLANE_ANGLE_UNIT()
SI_UNIT($,.RADIAN.)
);
#1606=(
NAMED_UNIT(*)
SI_UNIT($,.STERADIAN.)
SOLID_ANGLE_UNIT()
);
#1608=SHAPE_DEFINITION_REPRESENTATION(#1617,#1634);
#1617=PRODUCT_DEFINITION_SHAPE('',$,#1644);
#1634=SHAPE_REPRESENTATION('',(#872),#1594);
#1642=PRODUCT_DEFINITION_CONTEXT('part definition',#1671,'design');
#1644=PRODUCT_DEFINITION('Wheel','Wheel',#1653,#1642);
#1653=PRODUCT_DEFINITION_FORMATION('',$,#1674);
#1671=APPLICATION_CONTEXT(
'Core Data for Automotive Mechanical Design Process');
#1672=PRODUCT_CONTEXT('part definition',#1671,'mechanical');
#1674=PRODUCT('Wheel','Wheel',$,(#1672));
#1683=PRESENTATION_STYLE_ASSIGNMENT((#1687));
#1687=SURFACE_STYLE_USAGE(.BOTH.,#1691);
#1691=SURFACE_SIDE_STYLE('',(#1695));
#1695=SURFACE_STYLE_FILL_AREA(#1699);
#1699=FILL_AREA_STYLE('Opaque(0,85,255)',(#1703));
#1703=FILL_AREA_STYLE_COLOUR('Opaque(0,85,255)',#1707);
#1707=COLOUR_RGB('Opaque(0,85,255)', 0.09019608, 0.27058824, 0.51372549);
ENDSEC;
END-ISO-10303-21;
